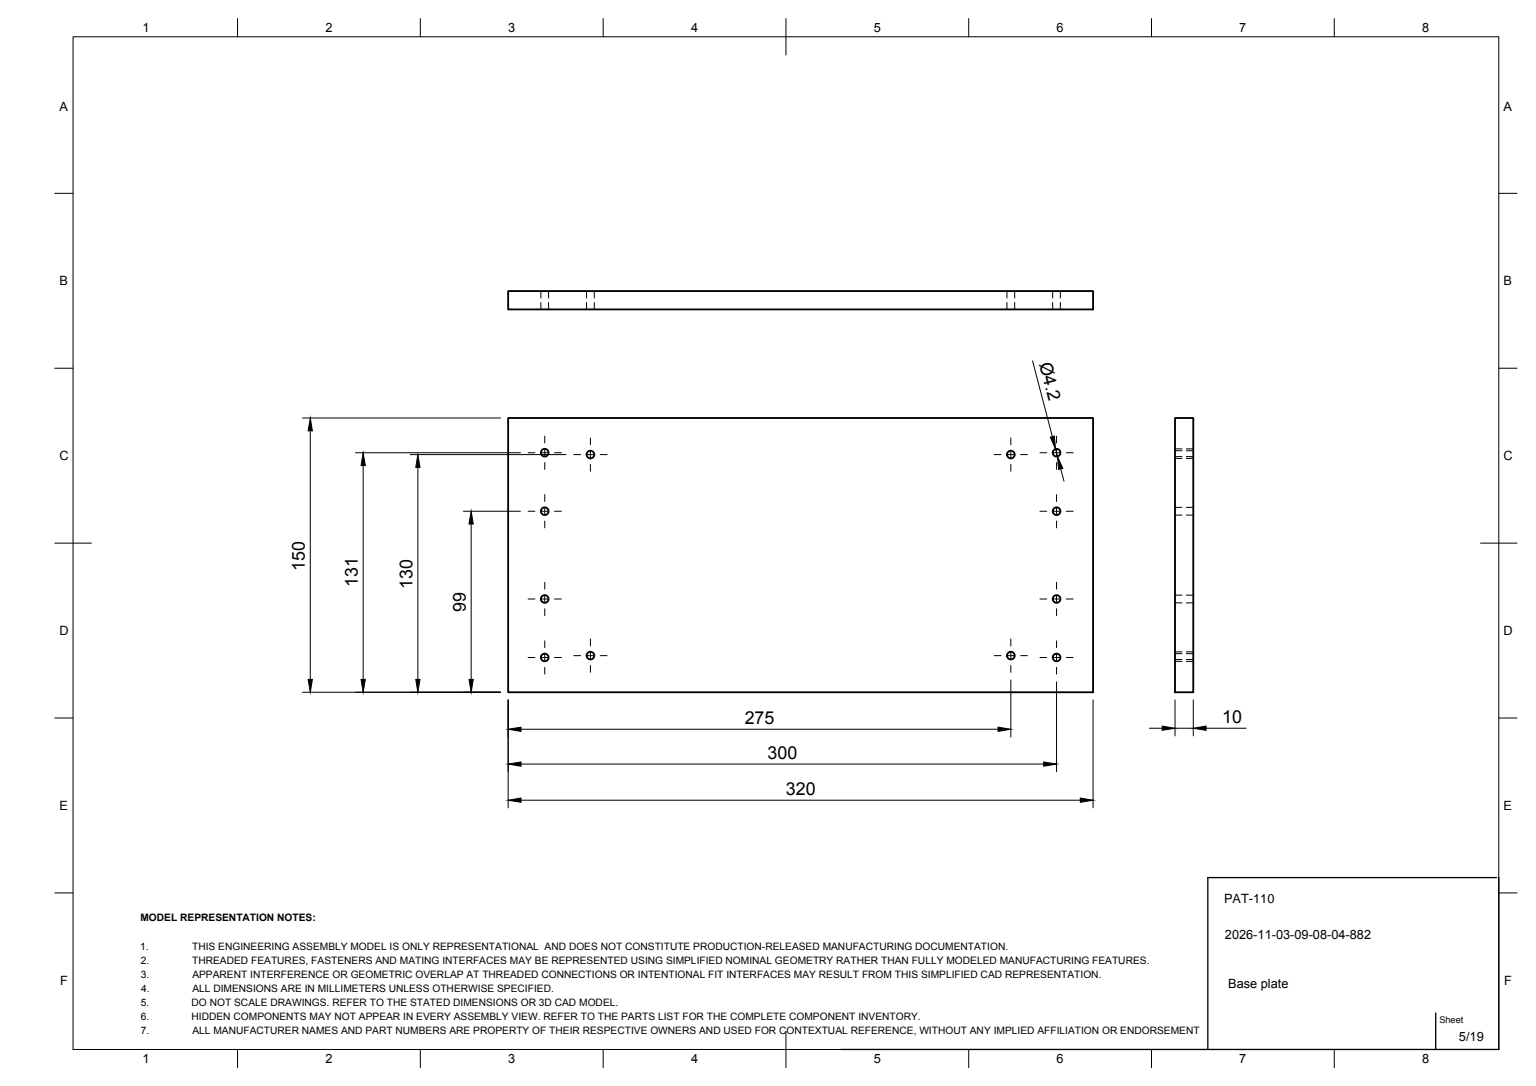
ISO-10303-21;
HEADER;
/* Generated by software containing ST-Developer
 * from STEP Tools, Inc. (www.steptools.com) 
 */

FILE_DESCRIPTION(
/* description */ ('Twin-shaft manual slide'),
/* implementation_level */ '2;1');

FILE_NAME(
/* name */ 'Base plate.step',
/* time_stamp */ '2026-10-27T18:38:08-07:00',
/* author */ (''),
/* organization */ (''),
/* preprocessor_version */ 'ST-DEVELOPER v20.2',
/* originating_system */ 'Autodesk Translation Framework v15.17.0.0',
/* authorisation */ '');

FILE_SCHEMA (('AUTOMOTIVE_DESIGN { 1 0 10303 214 3 1 1 }'));
ENDSEC;

DATA;
#10=MECHANICAL_DESIGN_GEOMETRIC_PRESENTATION_REPRESENTATION('',(#276),#6463);
#244=SHAPE_REPRESENTATION_RELATIONSHIP('SRR','None',#6562,#260);
#260=ADVANCED_BREP_SHAPE_REPRESENTATION('',(#292),#6445);
#276=STYLED_ITEM('',(#6719),#292);
#292=MANIFOLD_SOLID_BREP('Body1',#3638);
#304=FACE_BOUND('',#750,.T.);
#305=FACE_BOUND('',#751,.T.);
#306=FACE_BOUND('',#752,.T.);
#307=FACE_BOUND('',#753,.T.);
#308=FACE_BOUND('',#754,.T.);
#309=FACE_BOUND('',#755,.T.);
#310=FACE_BOUND('',#756,.T.);
#311=FACE_BOUND('',#757,.T.);
#312=FACE_BOUND('',#758,.T.);
#313=FACE_BOUND('',#759,.T.);
#314=FACE_BOUND('',#760,.T.);
#315=FACE_BOUND('',#761,.T.);
#316=FACE_BOUND('',#763,.T.);
#317=FACE_BOUND('',#764,.T.);
#318=FACE_BOUND('',#765,.T.);
#319=FACE_BOUND('',#766,.T.);
#320=FACE_BOUND('',#767,.T.);
#321=FACE_BOUND('',#768,.T.);
#322=FACE_BOUND('',#769,.T.);
#323=FACE_BOUND('',#770,.T.);
#324=FACE_BOUND('',#771,.T.);
#325=FACE_BOUND('',#772,.T.);
#326=FACE_BOUND('',#773,.T.);
#327=FACE_BOUND('',#774,.T.);
#401=PLANE('',#3874);
#402=PLANE('',#3875);
#403=PLANE('',#3876);
#404=PLANE('',#3877);
#405=PLANE('',#3878);
#406=PLANE('',#3879);
#526=FACE_OUTER_BOUND('',#733,.T.);
#527=FACE_OUTER_BOUND('',#734,.T.);
#528=FACE_OUTER_BOUND('',#735,.T.);
#529=FACE_OUTER_BOUND('',#736,.T.);
#530=FACE_OUTER_BOUND('',#737,.T.);
#531=FACE_OUTER_BOUND('',#738,.T.);
#532=FACE_OUTER_BOUND('',#739,.T.);
#533=FACE_OUTER_BOUND('',#740,.T.);
#534=FACE_OUTER_BOUND('',#741,.T.);
#535=FACE_OUTER_BOUND('',#742,.T.);
#536=FACE_OUTER_BOUND('',#743,.T.);
#537=FACE_OUTER_BOUND('',#744,.T.);
#538=FACE_OUTER_BOUND('',#745,.T.);
#539=FACE_OUTER_BOUND('',#746,.T.);
#540=FACE_OUTER_BOUND('',#747,.T.);
#541=FACE_OUTER_BOUND('',#748,.T.);
#542=FACE_OUTER_BOUND('',#749,.T.);
#543=FACE_OUTER_BOUND('',#762,.T.);
#733=EDGE_LOOP('',(#2488,#2489,#2490,#2491));
#734=EDGE_LOOP('',(#2492,#2493,#2494,#2495));
#735=EDGE_LOOP('',(#2496,#2497,#2498,#2499));
#736=EDGE_LOOP('',(#2500,#2501,#2502,#2503));
#737=EDGE_LOOP('',(#2504,#2505,#2506,#2507));
#738=EDGE_LOOP('',(#2508,#2509,#2510,#2511));
#739=EDGE_LOOP('',(#2512,#2513,#2514,#2515));
#740=EDGE_LOOP('',(#2516,#2517,#2518,#2519));
#741=EDGE_LOOP('',(#2520,#2521,#2522,#2523));
#742=EDGE_LOOP('',(#2524,#2525,#2526,#2527));
#743=EDGE_LOOP('',(#2528,#2529,#2530,#2531));
#744=EDGE_LOOP('',(#2532,#2533,#2534,#2535));
#745=EDGE_LOOP('',(#2536,#2537,#2538,#2539));
#746=EDGE_LOOP('',(#2540,#2541,#2542,#2543));
#747=EDGE_LOOP('',(#2544,#2545,#2546,#2547));
#748=EDGE_LOOP('',(#2548,#2549,#2550,#2551));
#749=EDGE_LOOP('',(#2552,#2553,#2554,#2555));
#750=EDGE_LOOP('',(#2556));
#751=EDGE_LOOP('',(#2557));
#752=EDGE_LOOP('',(#2558));
#753=EDGE_LOOP('',(#2559));
#754=EDGE_LOOP('',(#2560));
#755=EDGE_LOOP('',(#2561));
#756=EDGE_LOOP('',(#2562));
#757=EDGE_LOOP('',(#2563));
#758=EDGE_LOOP('',(#2564));
#759=EDGE_LOOP('',(#2565));
#760=EDGE_LOOP('',(#2566));
#761=EDGE_LOOP('',(#2567));
#762=EDGE_LOOP('',(#2568,#2569,#2570,#2571));
#763=EDGE_LOOP('',(#2572));
#764=EDGE_LOOP('',(#2573));
#765=EDGE_LOOP('',(#2574));
#766=EDGE_LOOP('',(#2575));
#767=EDGE_LOOP('',(#2576));
#768=EDGE_LOOP('',(#2577));
#769=EDGE_LOOP('',(#2578));
#770=EDGE_LOOP('',(#2579));
#771=EDGE_LOOP('',(#2580));
#772=EDGE_LOOP('',(#2581));
#773=EDGE_LOOP('',(#2582));
#774=EDGE_LOOP('',(#2583));
#1037=LINE('',#5424,#1323);
#1038=LINE('',#5430,#1324);
#1039=LINE('',#5436,#1325);
#1040=LINE('',#5442,#1326);
#1041=LINE('',#5448,#1327);
#1042=LINE('',#5454,#1328);
#1043=LINE('',#5460,#1329);
#1044=LINE('',#5466,#1330);
#1045=LINE('',#5472,#1331);
#1046=LINE('',#5478,#1332);
#1047=LINE('',#5484,#1333);
#1048=LINE('',#5490,#1334);
#1049=LINE('',#5495,#1335);
#1050=LINE('',#5497,#1336);
#1051=LINE('',#5499,#1337);
#1052=LINE('',#5500,#1338);
#1053=LINE('',#5503,#1339);
#1054=LINE('',#5505,#1340);
#1055=LINE('',#5506,#1341);
#1056=LINE('',#5509,#1342);
#1057=LINE('',#5511,#1343);
#1058=LINE('',#5512,#1344);
#1059=LINE('',#5514,#1345);
#1060=LINE('',#5515,#1346);
#1323=VECTOR('',#4277,0.210000000000001);
#1324=VECTOR('',#4284,0.21);
#1325=VECTOR('',#4291,0.21);
#1326=VECTOR('',#4298,0.210000000000001);
#1327=VECTOR('',#4305,0.210000000000001);
#1328=VECTOR('',#4312,0.210000000000001);
#1329=VECTOR('',#4319,0.21);
#1330=VECTOR('',#4326,0.21);
#1331=VECTOR('',#4333,0.21);
#1332=VECTOR('',#4340,0.21);
#1333=VECTOR('',#4347,0.210000000000001);
#1334=VECTOR('',#4354,0.210000000000001);
#1335=VECTOR('',#4359,1.);
#1336=VECTOR('',#4360,1.);
#1337=VECTOR('',#4361,1.);
#1338=VECTOR('',#4362,1.);
#1339=VECTOR('',#4365,1.);
#1340=VECTOR('',#4366,1.);
#1341=VECTOR('',#4367,1.);
#1342=VECTOR('',#4370,1.);
#1343=VECTOR('',#4371,1.);
#1344=VECTOR('',#4372,1.);
#1345=VECTOR('',#4375,1.);
#1346=VECTOR('',#4376,1.);
#1609=CIRCLE('',#3839,0.210000000000001);
#1610=CIRCLE('',#3840,0.210000000000001);
#1611=CIRCLE('',#3842,0.21);
#1612=CIRCLE('',#3843,0.21);
#1613=CIRCLE('',#3845,0.21);
#1614=CIRCLE('',#3846,0.21);
#1615=CIRCLE('',#3848,0.210000000000001);
#1616=CIRCLE('',#3849,0.210000000000001);
#1617=CIRCLE('',#3851,0.210000000000001);
#1618=CIRCLE('',#3852,0.210000000000001);
#1619=CIRCLE('',#3854,0.210000000000001);
#1620=CIRCLE('',#3855,0.210000000000001);
#1621=CIRCLE('',#3857,0.21);
#1622=CIRCLE('',#3858,0.21);
#1623=CIRCLE('',#3860,0.21);
#1624=CIRCLE('',#3861,0.21);
#1625=CIRCLE('',#3863,0.21);
#1626=CIRCLE('',#3864,0.21);
#1627=CIRCLE('',#3866,0.21);
#1628=CIRCLE('',#3867,0.21);
#1629=CIRCLE('',#3869,0.210000000000001);
#1630=CIRCLE('',#3870,0.210000000000001);
#1631=CIRCLE('',#3872,0.210000000000001);
#1632=CIRCLE('',#3873,0.210000000000001);
#1762=VERTEX_POINT('',#5421);
#1763=VERTEX_POINT('',#5423);
#1764=VERTEX_POINT('',#5427);
#1765=VERTEX_POINT('',#5429);
#1766=VERTEX_POINT('',#5433);
#1767=VERTEX_POINT('',#5435);
#1768=VERTEX_POINT('',#5439);
#1769=VERTEX_POINT('',#5441);
#1770=VERTEX_POINT('',#5445);
#1771=VERTEX_POINT('',#5447);
#1772=VERTEX_POINT('',#5451);
#1773=VERTEX_POINT('',#5453);
#1774=VERTEX_POINT('',#5457);
#1775=VERTEX_POINT('',#5459);
#1776=VERTEX_POINT('',#5463);
#1777=VERTEX_POINT('',#5465);
#1778=VERTEX_POINT('',#5469);
#1779=VERTEX_POINT('',#5471);
#1780=VERTEX_POINT('',#5475);
#1781=VERTEX_POINT('',#5477);
#1782=VERTEX_POINT('',#5481);
#1783=VERTEX_POINT('',#5483);
#1784=VERTEX_POINT('',#5487);
#1785=VERTEX_POINT('',#5489);
#1786=VERTEX_POINT('',#5493);
#1787=VERTEX_POINT('',#5494);
#1788=VERTEX_POINT('',#5496);
#1789=VERTEX_POINT('',#5498);
#1790=VERTEX_POINT('',#5502);
#1791=VERTEX_POINT('',#5504);
#1792=VERTEX_POINT('',#5508);
#1793=VERTEX_POINT('',#5510);
#2049=EDGE_CURVE('',#1762,#1762,#1609,.T.);
#2050=EDGE_CURVE('',#1762,#1763,#1037,.T.);
#2051=EDGE_CURVE('',#1763,#1763,#1610,.T.);
#2052=EDGE_CURVE('',#1764,#1764,#1611,.T.);
#2053=EDGE_CURVE('',#1764,#1765,#1038,.T.);
#2054=EDGE_CURVE('',#1765,#1765,#1612,.T.);
#2055=EDGE_CURVE('',#1766,#1766,#1613,.T.);
#2056=EDGE_CURVE('',#1766,#1767,#1039,.T.);
#2057=EDGE_CURVE('',#1767,#1767,#1614,.T.);
#2058=EDGE_CURVE('',#1768,#1768,#1615,.T.);
#2059=EDGE_CURVE('',#1768,#1769,#1040,.T.);
#2060=EDGE_CURVE('',#1769,#1769,#1616,.T.);
#2061=EDGE_CURVE('',#1770,#1770,#1617,.T.);
#2062=EDGE_CURVE('',#1770,#1771,#1041,.T.);
#2063=EDGE_CURVE('',#1771,#1771,#1618,.T.);
#2064=EDGE_CURVE('',#1772,#1772,#1619,.T.);
#2065=EDGE_CURVE('',#1772,#1773,#1042,.T.);
#2066=EDGE_CURVE('',#1773,#1773,#1620,.T.);
#2067=EDGE_CURVE('',#1774,#1774,#1621,.T.);
#2068=EDGE_CURVE('',#1774,#1775,#1043,.T.);
#2069=EDGE_CURVE('',#1775,#1775,#1622,.T.);
#2070=EDGE_CURVE('',#1776,#1776,#1623,.T.);
#2071=EDGE_CURVE('',#1776,#1777,#1044,.T.);
#2072=EDGE_CURVE('',#1777,#1777,#1624,.T.);
#2073=EDGE_CURVE('',#1778,#1778,#1625,.T.);
#2074=EDGE_CURVE('',#1778,#1779,#1045,.T.);
#2075=EDGE_CURVE('',#1779,#1779,#1626,.T.);
#2076=EDGE_CURVE('',#1780,#1780,#1627,.T.);
#2077=EDGE_CURVE('',#1780,#1781,#1046,.T.);
#2078=EDGE_CURVE('',#1781,#1781,#1628,.T.);
#2079=EDGE_CURVE('',#1782,#1782,#1629,.T.);
#2080=EDGE_CURVE('',#1782,#1783,#1047,.T.);
#2081=EDGE_CURVE('',#1783,#1783,#1630,.T.);
#2082=EDGE_CURVE('',#1784,#1784,#1631,.T.);
#2083=EDGE_CURVE('',#1784,#1785,#1048,.T.);
#2084=EDGE_CURVE('',#1785,#1785,#1632,.T.);
#2085=EDGE_CURVE('',#1786,#1787,#1049,.T.);
#2086=EDGE_CURVE('',#1787,#1788,#1050,.T.);
#2087=EDGE_CURVE('',#1789,#1788,#1051,.T.);
#2088=EDGE_CURVE('',#1786,#1789,#1052,.T.);
#2089=EDGE_CURVE('',#1790,#1786,#1053,.T.);
#2090=EDGE_CURVE('',#1791,#1789,#1054,.T.);
#2091=EDGE_CURVE('',#1790,#1791,#1055,.T.);
#2092=EDGE_CURVE('',#1792,#1790,#1056,.T.);
#2093=EDGE_CURVE('',#1793,#1791,#1057,.T.);
#2094=EDGE_CURVE('',#1792,#1793,#1058,.T.);
#2095=EDGE_CURVE('',#1787,#1792,#1059,.T.);
#2096=EDGE_CURVE('',#1788,#1793,#1060,.T.);
#2488=ORIENTED_EDGE('',*,*,#2049,.F.);
#2489=ORIENTED_EDGE('',*,*,#2050,.T.);
#2490=ORIENTED_EDGE('',*,*,#2051,.F.);
#2491=ORIENTED_EDGE('',*,*,#2050,.F.);
#2492=ORIENTED_EDGE('',*,*,#2052,.F.);
#2493=ORIENTED_EDGE('',*,*,#2053,.T.);
#2494=ORIENTED_EDGE('',*,*,#2054,.F.);
#2495=ORIENTED_EDGE('',*,*,#2053,.F.);
#2496=ORIENTED_EDGE('',*,*,#2055,.F.);
#2497=ORIENTED_EDGE('',*,*,#2056,.T.);
#2498=ORIENTED_EDGE('',*,*,#2057,.F.);
#2499=ORIENTED_EDGE('',*,*,#2056,.F.);
#2500=ORIENTED_EDGE('',*,*,#2058,.F.);
#2501=ORIENTED_EDGE('',*,*,#2059,.T.);
#2502=ORIENTED_EDGE('',*,*,#2060,.F.);
#2503=ORIENTED_EDGE('',*,*,#2059,.F.);
#2504=ORIENTED_EDGE('',*,*,#2061,.F.);
#2505=ORIENTED_EDGE('',*,*,#2062,.T.);
#2506=ORIENTED_EDGE('',*,*,#2063,.F.);
#2507=ORIENTED_EDGE('',*,*,#2062,.F.);
#2508=ORIENTED_EDGE('',*,*,#2064,.F.);
#2509=ORIENTED_EDGE('',*,*,#2065,.T.);
#2510=ORIENTED_EDGE('',*,*,#2066,.F.);
#2511=ORIENTED_EDGE('',*,*,#2065,.F.);
#2512=ORIENTED_EDGE('',*,*,#2067,.F.);
#2513=ORIENTED_EDGE('',*,*,#2068,.T.);
#2514=ORIENTED_EDGE('',*,*,#2069,.F.);
#2515=ORIENTED_EDGE('',*,*,#2068,.F.);
#2516=ORIENTED_EDGE('',*,*,#2070,.F.);
#2517=ORIENTED_EDGE('',*,*,#2071,.T.);
#2518=ORIENTED_EDGE('',*,*,#2072,.F.);
#2519=ORIENTED_EDGE('',*,*,#2071,.F.);
#2520=ORIENTED_EDGE('',*,*,#2073,.F.);
#2521=ORIENTED_EDGE('',*,*,#2074,.T.);
#2522=ORIENTED_EDGE('',*,*,#2075,.F.);
#2523=ORIENTED_EDGE('',*,*,#2074,.F.);
#2524=ORIENTED_EDGE('',*,*,#2076,.F.);
#2525=ORIENTED_EDGE('',*,*,#2077,.T.);
#2526=ORIENTED_EDGE('',*,*,#2078,.F.);
#2527=ORIENTED_EDGE('',*,*,#2077,.F.);
#2528=ORIENTED_EDGE('',*,*,#2079,.F.);
#2529=ORIENTED_EDGE('',*,*,#2080,.T.);
#2530=ORIENTED_EDGE('',*,*,#2081,.F.);
#2531=ORIENTED_EDGE('',*,*,#2080,.F.);
#2532=ORIENTED_EDGE('',*,*,#2082,.F.);
#2533=ORIENTED_EDGE('',*,*,#2083,.T.);
#2534=ORIENTED_EDGE('',*,*,#2084,.F.);
#2535=ORIENTED_EDGE('',*,*,#2083,.F.);
#2536=ORIENTED_EDGE('',*,*,#2085,.T.);
#2537=ORIENTED_EDGE('',*,*,#2086,.T.);
#2538=ORIENTED_EDGE('',*,*,#2087,.F.);
#2539=ORIENTED_EDGE('',*,*,#2088,.F.);
#2540=ORIENTED_EDGE('',*,*,#2089,.T.);
#2541=ORIENTED_EDGE('',*,*,#2088,.T.);
#2542=ORIENTED_EDGE('',*,*,#2090,.F.);
#2543=ORIENTED_EDGE('',*,*,#2091,.F.);
#2544=ORIENTED_EDGE('',*,*,#2092,.T.);
#2545=ORIENTED_EDGE('',*,*,#2091,.T.);
#2546=ORIENTED_EDGE('',*,*,#2093,.F.);
#2547=ORIENTED_EDGE('',*,*,#2094,.F.);
#2548=ORIENTED_EDGE('',*,*,#2095,.T.);
#2549=ORIENTED_EDGE('',*,*,#2094,.T.);
#2550=ORIENTED_EDGE('',*,*,#2096,.F.);
#2551=ORIENTED_EDGE('',*,*,#2086,.F.);
#2552=ORIENTED_EDGE('',*,*,#2096,.T.);
#2553=ORIENTED_EDGE('',*,*,#2093,.T.);
#2554=ORIENTED_EDGE('',*,*,#2090,.T.);
#2555=ORIENTED_EDGE('',*,*,#2087,.T.);
#2556=ORIENTED_EDGE('',*,*,#2063,.T.);
#2557=ORIENTED_EDGE('',*,*,#2066,.T.);
#2558=ORIENTED_EDGE('',*,*,#2069,.T.);
#2559=ORIENTED_EDGE('',*,*,#2072,.T.);
#2560=ORIENTED_EDGE('',*,*,#2075,.T.);
#2561=ORIENTED_EDGE('',*,*,#2078,.T.);
#2562=ORIENTED_EDGE('',*,*,#2081,.T.);
#2563=ORIENTED_EDGE('',*,*,#2084,.T.);
#2564=ORIENTED_EDGE('',*,*,#2060,.T.);
#2565=ORIENTED_EDGE('',*,*,#2057,.T.);
#2566=ORIENTED_EDGE('',*,*,#2054,.T.);
#2567=ORIENTED_EDGE('',*,*,#2051,.T.);
#2568=ORIENTED_EDGE('',*,*,#2095,.F.);
#2569=ORIENTED_EDGE('',*,*,#2085,.F.);
#2570=ORIENTED_EDGE('',*,*,#2089,.F.);
#2571=ORIENTED_EDGE('',*,*,#2092,.F.);
#2572=ORIENTED_EDGE('',*,*,#2061,.T.);
#2573=ORIENTED_EDGE('',*,*,#2064,.T.);
#2574=ORIENTED_EDGE('',*,*,#2067,.T.);
#2575=ORIENTED_EDGE('',*,*,#2070,.T.);
#2576=ORIENTED_EDGE('',*,*,#2073,.T.);
#2577=ORIENTED_EDGE('',*,*,#2076,.T.);
#2578=ORIENTED_EDGE('',*,*,#2079,.T.);
#2579=ORIENTED_EDGE('',*,*,#2082,.T.);
#2580=ORIENTED_EDGE('',*,*,#2058,.T.);
#2581=ORIENTED_EDGE('',*,*,#2055,.T.);
#2582=ORIENTED_EDGE('',*,*,#2052,.T.);
#2583=ORIENTED_EDGE('',*,*,#2049,.T.);
#3366=CYLINDRICAL_SURFACE('',#3838,0.210000000000001);
#3367=CYLINDRICAL_SURFACE('',#3841,0.21);
#3368=CYLINDRICAL_SURFACE('',#3844,0.21);
#3369=CYLINDRICAL_SURFACE('',#3847,0.210000000000001);
#3370=CYLINDRICAL_SURFACE('',#3850,0.210000000000001);
#3371=CYLINDRICAL_SURFACE('',#3853,0.210000000000001);
#3372=CYLINDRICAL_SURFACE('',#3856,0.21);
#3373=CYLINDRICAL_SURFACE('',#3859,0.21);
#3374=CYLINDRICAL_SURFACE('',#3862,0.21);
#3375=CYLINDRICAL_SURFACE('',#3865,0.21);
#3376=CYLINDRICAL_SURFACE('',#3868,0.210000000000001);
#3377=CYLINDRICAL_SURFACE('',#3871,0.210000000000001);
#3431=ADVANCED_FACE('',(#526),#3366,.F.);
#3432=ADVANCED_FACE('',(#527),#3367,.F.);
#3433=ADVANCED_FACE('',(#528),#3368,.F.);
#3434=ADVANCED_FACE('',(#529),#3369,.F.);
#3435=ADVANCED_FACE('',(#530),#3370,.F.);
#3436=ADVANCED_FACE('',(#531),#3371,.F.);
#3437=ADVANCED_FACE('',(#532),#3372,.F.);
#3438=ADVANCED_FACE('',(#533),#3373,.F.);
#3439=ADVANCED_FACE('',(#534),#3374,.F.);
#3440=ADVANCED_FACE('',(#535),#3375,.F.);
#3441=ADVANCED_FACE('',(#536),#3376,.F.);
#3442=ADVANCED_FACE('',(#537),#3377,.F.);
#3443=ADVANCED_FACE('',(#538),#401,.T.);
#3444=ADVANCED_FACE('',(#539),#402,.T.);
#3445=ADVANCED_FACE('',(#540),#403,.T.);
#3446=ADVANCED_FACE('',(#541),#404,.T.);
#3447=ADVANCED_FACE('',(#542,#304,#305,#306,#307,#308,#309,#310,#311,#312,
#313,#314,#315),#405,.T.);
#3448=ADVANCED_FACE('',(#543,#316,#317,#318,#319,#320,#321,#322,#323,#324,
#325,#326,#327),#406,.F.);
#3638=CLOSED_SHELL('',(#3431,#3432,#3433,#3434,#3435,#3436,#3437,#3438,
#3439,#3440,#3441,#3442,#3443,#3444,#3445,#3446,#3447,#3448));
#3837=AXIS2_PLACEMENT_3D('',#5419,#4271,#4272);
#3838=AXIS2_PLACEMENT_3D('',#5420,#4273,#4274);
#3839=AXIS2_PLACEMENT_3D('',#5422,#4275,#4276);
#3840=AXIS2_PLACEMENT_3D('',#5425,#4278,#4279);
#3841=AXIS2_PLACEMENT_3D('',#5426,#4280,#4281);
#3842=AXIS2_PLACEMENT_3D('',#5428,#4282,#4283);
#3843=AXIS2_PLACEMENT_3D('',#5431,#4285,#4286);
#3844=AXIS2_PLACEMENT_3D('',#5432,#4287,#4288);
#3845=AXIS2_PLACEMENT_3D('',#5434,#4289,#4290);
#3846=AXIS2_PLACEMENT_3D('',#5437,#4292,#4293);
#3847=AXIS2_PLACEMENT_3D('',#5438,#4294,#4295);
#3848=AXIS2_PLACEMENT_3D('',#5440,#4296,#4297);
#3849=AXIS2_PLACEMENT_3D('',#5443,#4299,#4300);
#3850=AXIS2_PLACEMENT_3D('',#5444,#4301,#4302);
#3851=AXIS2_PLACEMENT_3D('',#5446,#4303,#4304);
#3852=AXIS2_PLACEMENT_3D('',#5449,#4306,#4307);
#3853=AXIS2_PLACEMENT_3D('',#5450,#4308,#4309);
#3854=AXIS2_PLACEMENT_3D('',#5452,#4310,#4311);
#3855=AXIS2_PLACEMENT_3D('',#5455,#4313,#4314);
#3856=AXIS2_PLACEMENT_3D('',#5456,#4315,#4316);
#3857=AXIS2_PLACEMENT_3D('',#5458,#4317,#4318);
#3858=AXIS2_PLACEMENT_3D('',#5461,#4320,#4321);
#3859=AXIS2_PLACEMENT_3D('',#5462,#4322,#4323);
#3860=AXIS2_PLACEMENT_3D('',#5464,#4324,#4325);
#3861=AXIS2_PLACEMENT_3D('',#5467,#4327,#4328);
#3862=AXIS2_PLACEMENT_3D('',#5468,#4329,#4330);
#3863=AXIS2_PLACEMENT_3D('',#5470,#4331,#4332);
#3864=AXIS2_PLACEMENT_3D('',#5473,#4334,#4335);
#3865=AXIS2_PLACEMENT_3D('',#5474,#4336,#4337);
#3866=AXIS2_PLACEMENT_3D('',#5476,#4338,#4339);
#3867=AXIS2_PLACEMENT_3D('',#5479,#4341,#4342);
#3868=AXIS2_PLACEMENT_3D('',#5480,#4343,#4344);
#3869=AXIS2_PLACEMENT_3D('',#5482,#4345,#4346);
#3870=AXIS2_PLACEMENT_3D('',#5485,#4348,#4349);
#3871=AXIS2_PLACEMENT_3D('',#5486,#4350,#4351);
#3872=AXIS2_PLACEMENT_3D('',#5488,#4352,#4353);
#3873=AXIS2_PLACEMENT_3D('',#5491,#4355,#4356);
#3874=AXIS2_PLACEMENT_3D('',#5492,#4357,#4358);
#3875=AXIS2_PLACEMENT_3D('',#5501,#4363,#4364);
#3876=AXIS2_PLACEMENT_3D('',#5507,#4368,#4369);
#3877=AXIS2_PLACEMENT_3D('',#5513,#4373,#4374);
#3878=AXIS2_PLACEMENT_3D('',#5516,#4377,#4378);
#3879=AXIS2_PLACEMENT_3D('',#5517,#4379,#4380);
#4271=DIRECTION('axis',(0.,0.,1.));
#4272=DIRECTION('refdir',(1.,0.,0.));
#4273=DIRECTION('center_axis',(0.,0.,1.));
#4274=DIRECTION('ref_axis',(1.,0.,0.));
#4275=DIRECTION('center_axis',(0.,0.,1.));
#4276=DIRECTION('ref_axis',(1.,0.,0.));
#4277=DIRECTION('',(0.,0.,1.));
#4278=DIRECTION('center_axis',(0.,0.,-1.));
#4279=DIRECTION('ref_axis',(1.,0.,0.));
#4280=DIRECTION('center_axis',(0.,0.,1.));
#4281=DIRECTION('ref_axis',(1.,0.,0.));
#4282=DIRECTION('center_axis',(0.,0.,1.));
#4283=DIRECTION('ref_axis',(1.,0.,0.));
#4284=DIRECTION('',(0.,0.,1.));
#4285=DIRECTION('center_axis',(0.,0.,-1.));
#4286=DIRECTION('ref_axis',(1.,0.,0.));
#4287=DIRECTION('center_axis',(0.,0.,1.));
#4288=DIRECTION('ref_axis',(1.,0.,0.));
#4289=DIRECTION('center_axis',(0.,0.,1.));
#4290=DIRECTION('ref_axis',(1.,0.,0.));
#4291=DIRECTION('',(0.,0.,1.));
#4292=DIRECTION('center_axis',(0.,0.,-1.));
#4293=DIRECTION('ref_axis',(1.,0.,0.));
#4294=DIRECTION('center_axis',(0.,0.,1.));
#4295=DIRECTION('ref_axis',(1.,0.,0.));
#4296=DIRECTION('center_axis',(0.,0.,1.));
#4297=DIRECTION('ref_axis',(1.,0.,0.));
#4298=DIRECTION('',(0.,0.,1.));
#4299=DIRECTION('center_axis',(0.,0.,-1.));
#4300=DIRECTION('ref_axis',(1.,0.,0.));
#4301=DIRECTION('center_axis',(0.,0.,1.));
#4302=DIRECTION('ref_axis',(1.,0.,0.));
#4303=DIRECTION('center_axis',(0.,0.,1.));
#4304=DIRECTION('ref_axis',(1.,0.,0.));
#4305=DIRECTION('',(0.,0.,1.));
#4306=DIRECTION('center_axis',(0.,0.,-1.));
#4307=DIRECTION('ref_axis',(1.,0.,0.));
#4308=DIRECTION('center_axis',(0.,0.,1.));
#4309=DIRECTION('ref_axis',(1.,0.,0.));
#4310=DIRECTION('center_axis',(0.,0.,1.));
#4311=DIRECTION('ref_axis',(1.,0.,0.));
#4312=DIRECTION('',(0.,0.,1.));
#4313=DIRECTION('center_axis',(0.,0.,-1.));
#4314=DIRECTION('ref_axis',(1.,0.,0.));
#4315=DIRECTION('center_axis',(0.,0.,1.));
#4316=DIRECTION('ref_axis',(1.,0.,0.));
#4317=DIRECTION('center_axis',(0.,0.,1.));
#4318=DIRECTION('ref_axis',(1.,0.,0.));
#4319=DIRECTION('',(0.,0.,1.));
#4320=DIRECTION('center_axis',(0.,0.,-1.));
#4321=DIRECTION('ref_axis',(1.,0.,0.));
#4322=DIRECTION('center_axis',(0.,0.,1.));
#4323=DIRECTION('ref_axis',(1.,0.,0.));
#4324=DIRECTION('center_axis',(0.,0.,1.));
#4325=DIRECTION('ref_axis',(1.,0.,0.));
#4326=DIRECTION('',(0.,0.,1.));
#4327=DIRECTION('center_axis',(0.,0.,-1.));
#4328=DIRECTION('ref_axis',(1.,0.,0.));
#4329=DIRECTION('center_axis',(0.,0.,1.));
#4330=DIRECTION('ref_axis',(1.,0.,0.));
#4331=DIRECTION('center_axis',(0.,0.,1.));
#4332=DIRECTION('ref_axis',(1.,0.,0.));
#4333=DIRECTION('',(0.,0.,1.));
#4334=DIRECTION('center_axis',(0.,0.,-1.));
#4335=DIRECTION('ref_axis',(1.,0.,0.));
#4336=DIRECTION('center_axis',(0.,0.,1.));
#4337=DIRECTION('ref_axis',(1.,0.,0.));
#4338=DIRECTION('center_axis',(0.,0.,1.));
#4339=DIRECTION('ref_axis',(1.,0.,0.));
#4340=DIRECTION('',(0.,0.,1.));
#4341=DIRECTION('center_axis',(0.,0.,-1.));
#4342=DIRECTION('ref_axis',(1.,0.,0.));
#4343=DIRECTION('center_axis',(0.,0.,1.));
#4344=DIRECTION('ref_axis',(1.,0.,0.));
#4345=DIRECTION('center_axis',(0.,0.,1.));
#4346=DIRECTION('ref_axis',(1.,0.,0.));
#4347=DIRECTION('',(0.,0.,1.));
#4348=DIRECTION('center_axis',(0.,0.,-1.));
#4349=DIRECTION('ref_axis',(1.,0.,0.));
#4350=DIRECTION('center_axis',(0.,0.,1.));
#4351=DIRECTION('ref_axis',(1.,0.,0.));
#4352=DIRECTION('center_axis',(0.,0.,1.));
#4353=DIRECTION('ref_axis',(1.,0.,0.));
#4354=DIRECTION('',(0.,0.,1.));
#4355=DIRECTION('center_axis',(0.,0.,-1.));
#4356=DIRECTION('ref_axis',(1.,0.,0.));
#4357=DIRECTION('center_axis',(0.,1.,0.));
#4358=DIRECTION('ref_axis',(-1.,0.,0.));
#4359=DIRECTION('',(-1.,0.,0.));
#4360=DIRECTION('',(0.,0.,1.));
#4361=DIRECTION('',(-1.,0.,0.));
#4362=DIRECTION('',(0.,0.,1.));
#4363=DIRECTION('center_axis',(1.,0.,0.));
#4364=DIRECTION('ref_axis',(0.,1.,0.));
#4365=DIRECTION('',(0.,1.,0.));
#4366=DIRECTION('',(0.,1.,0.));
#4367=DIRECTION('',(0.,0.,1.));
#4368=DIRECTION('center_axis',(0.,-1.,0.));
#4369=DIRECTION('ref_axis',(1.,0.,0.));
#4370=DIRECTION('',(1.,0.,0.));
#4371=DIRECTION('',(1.,0.,0.));
#4372=DIRECTION('',(0.,0.,1.));
#4373=DIRECTION('center_axis',(-1.,0.,0.));
#4374=DIRECTION('ref_axis',(0.,-1.,0.));
#4375=DIRECTION('',(0.,-1.,0.));
#4376=DIRECTION('',(0.,-1.,0.));
#4377=DIRECTION('center_axis',(0.,0.,1.));
#4378=DIRECTION('ref_axis',(1.,0.,0.));
#4379=DIRECTION('center_axis',(0.,0.,1.));
#4380=DIRECTION('ref_axis',(1.,0.,0.));
#5419=CARTESIAN_POINT('',(0.,0.,0.));
#5420=CARTESIAN_POINT('Origin',(26.5,-5.5,-0.1));
#5421=CARTESIAN_POINT('',(26.29,-5.5,0.));
#5422=CARTESIAN_POINT('Origin',(26.5,-5.5,0.));
#5423=CARTESIAN_POINT('',(26.29,-5.5,1.));
#5424=CARTESIAN_POINT('',(26.29,-5.5,-0.1));
#5425=CARTESIAN_POINT('Origin',(26.5,-5.5,1.));
#5426=CARTESIAN_POINT('Origin',(3.5,5.5,-0.1));
#5427=CARTESIAN_POINT('',(3.29,5.5,0.));
#5428=CARTESIAN_POINT('Origin',(3.5,5.5,0.));
#5429=CARTESIAN_POINT('',(3.29,5.5,1.));
#5430=CARTESIAN_POINT('',(3.29,5.5,-0.1));
#5431=CARTESIAN_POINT('Origin',(3.5,5.5,1.));
#5432=CARTESIAN_POINT('Origin',(3.5,-5.5,-0.1));
#5433=CARTESIAN_POINT('',(3.29,-5.5,0.));
#5434=CARTESIAN_POINT('Origin',(3.5,-5.5,0.));
#5435=CARTESIAN_POINT('',(3.29,-5.5,1.));
#5436=CARTESIAN_POINT('',(3.29,-5.5,-0.1));
#5437=CARTESIAN_POINT('Origin',(3.5,-5.5,1.));
#5438=CARTESIAN_POINT('Origin',(26.5,5.5,-0.1));
#5439=CARTESIAN_POINT('',(26.29,5.5,0.));
#5440=CARTESIAN_POINT('Origin',(26.5,5.5,0.));
#5441=CARTESIAN_POINT('',(26.29,5.5,1.));
#5442=CARTESIAN_POINT('',(26.29,5.5,-0.1));
#5443=CARTESIAN_POINT('Origin',(26.5,5.5,1.));
#5444=CARTESIAN_POINT('Origin',(29.,2.4,-0.1));
#5445=CARTESIAN_POINT('',(28.79,2.4,0.));
#5446=CARTESIAN_POINT('Origin',(29.,2.4,0.));
#5447=CARTESIAN_POINT('',(28.79,2.4,1.));
#5448=CARTESIAN_POINT('',(28.79,2.4,-0.1));
#5449=CARTESIAN_POINT('Origin',(29.,2.4,1.));
#5450=CARTESIAN_POINT('Origin',(29.,-5.6,-0.1));
#5451=CARTESIAN_POINT('',(28.79,-5.6,0.));
#5452=CARTESIAN_POINT('Origin',(29.,-5.6,0.));
#5453=CARTESIAN_POINT('',(28.79,-5.6,1.));
#5454=CARTESIAN_POINT('',(28.79,-5.6,-0.1));
#5455=CARTESIAN_POINT('Origin',(29.,-5.6,1.));
#5456=CARTESIAN_POINT('Origin',(1.,5.6,-0.1));
#5457=CARTESIAN_POINT('',(0.79,5.6,0.));
#5458=CARTESIAN_POINT('Origin',(1.,5.6,0.));
#5459=CARTESIAN_POINT('',(0.79,5.6,1.));
#5460=CARTESIAN_POINT('',(0.79,5.6,-0.1));
#5461=CARTESIAN_POINT('Origin',(1.,5.6,1.));
#5462=CARTESIAN_POINT('Origin',(1.,-2.4,-0.1));
#5463=CARTESIAN_POINT('',(0.79,-2.4,0.));
#5464=CARTESIAN_POINT('Origin',(1.,-2.4,0.));
#5465=CARTESIAN_POINT('',(0.79,-2.4,1.));
#5466=CARTESIAN_POINT('',(0.79,-2.4,-0.1));
#5467=CARTESIAN_POINT('Origin',(1.,-2.4,1.));
#5468=CARTESIAN_POINT('Origin',(1.,2.4,-0.1));
#5469=CARTESIAN_POINT('',(0.79,2.4,0.));
#5470=CARTESIAN_POINT('Origin',(1.,2.4,0.));
#5471=CARTESIAN_POINT('',(0.79,2.4,1.));
#5472=CARTESIAN_POINT('',(0.79,2.4,-0.1));
#5473=CARTESIAN_POINT('Origin',(1.,2.4,1.));
#5474=CARTESIAN_POINT('Origin',(1.,-5.6,-0.1));
#5475=CARTESIAN_POINT('',(0.79,-5.6,0.));
#5476=CARTESIAN_POINT('Origin',(1.,-5.6,0.));
#5477=CARTESIAN_POINT('',(0.79,-5.6,1.));
#5478=CARTESIAN_POINT('',(0.79,-5.6,-0.1));
#5479=CARTESIAN_POINT('Origin',(1.,-5.6,1.));
#5480=CARTESIAN_POINT('Origin',(29.,-2.4,-0.1));
#5481=CARTESIAN_POINT('',(28.79,-2.4,0.));
#5482=CARTESIAN_POINT('Origin',(29.,-2.4,0.));
#5483=CARTESIAN_POINT('',(28.79,-2.4,1.));
#5484=CARTESIAN_POINT('',(28.79,-2.4,-0.1));
#5485=CARTESIAN_POINT('Origin',(29.,-2.4,1.));
#5486=CARTESIAN_POINT('Origin',(29.,5.6,-0.1));
#5487=CARTESIAN_POINT('',(28.79,5.6,0.));
#5488=CARTESIAN_POINT('Origin',(29.,5.6,0.));
#5489=CARTESIAN_POINT('',(28.79,5.6,1.));
#5490=CARTESIAN_POINT('',(28.79,5.6,-0.1));
#5491=CARTESIAN_POINT('Origin',(29.,5.6,1.));
#5492=CARTESIAN_POINT('Origin',(31.,7.5,0.));
#5493=CARTESIAN_POINT('',(31.,7.5,0.));
#5494=CARTESIAN_POINT('',(-1.,7.5,0.));
#5495=CARTESIAN_POINT('',(31.,7.5,0.));
#5496=CARTESIAN_POINT('',(-1.,7.5,1.));
#5497=CARTESIAN_POINT('',(-1.,7.5,0.));
#5498=CARTESIAN_POINT('',(31.,7.5,1.));
#5499=CARTESIAN_POINT('',(31.,7.5,1.));
#5500=CARTESIAN_POINT('',(31.,7.5,0.));
#5501=CARTESIAN_POINT('Origin',(31.,-7.5,0.));
#5502=CARTESIAN_POINT('',(31.,-7.5,0.));
#5503=CARTESIAN_POINT('',(31.,-7.5,0.));
#5504=CARTESIAN_POINT('',(31.,-7.5,1.));
#5505=CARTESIAN_POINT('',(31.,-7.5,1.));
#5506=CARTESIAN_POINT('',(31.,-7.5,0.));
#5507=CARTESIAN_POINT('Origin',(-1.,-7.5,0.));
#5508=CARTESIAN_POINT('',(-1.,-7.5,0.));
#5509=CARTESIAN_POINT('',(-1.,-7.5,0.));
#5510=CARTESIAN_POINT('',(-1.,-7.5,1.));
#5511=CARTESIAN_POINT('',(-1.,-7.5,1.));
#5512=CARTESIAN_POINT('',(-1.,-7.5,0.));
#5513=CARTESIAN_POINT('Origin',(-1.,7.5,0.));
#5514=CARTESIAN_POINT('',(-1.,7.5,0.));
#5515=CARTESIAN_POINT('',(-1.,7.5,1.));
#5516=CARTESIAN_POINT('Origin',(15.,0.,1.));
#5517=CARTESIAN_POINT('Origin',(15.,0.,0.));
#6424=UNCERTAINTY_MEASURE_WITH_UNIT(LENGTH_MEASURE(0.001),#6464,
'DISTANCE_ACCURACY_VALUE',
'Maximum model space distance between geometric entities at asserted c
onnectivities');
#6442=UNCERTAINTY_MEASURE_WITH_UNIT(LENGTH_MEASURE(0.001),#6464,
'DISTANCE_ACCURACY_VALUE',
'Maximum model space distance between geometric entities at asserted c
onnectivities');
#6445=(
GEOMETRIC_REPRESENTATION_CONTEXT(3)
GLOBAL_UNCERTAINTY_ASSIGNED_CONTEXT((#6424))
GLOBAL_UNIT_ASSIGNED_CONTEXT((#6464,#6466,#6467))
REPRESENTATION_CONTEXT('','3D')
);
#6463=(
GEOMETRIC_REPRESENTATION_CONTEXT(3)
GLOBAL_UNCERTAINTY_ASSIGNED_CONTEXT((#6442))
GLOBAL_UNIT_ASSIGNED_CONTEXT((#6464,#6466,#6467))
REPRESENTATION_CONTEXT('','3D')
);
#6464=(
LENGTH_UNIT()
NAMED_UNIT(*)
SI_UNIT(.CENTI.,.METRE.)
);
#6466=(
NAMED_UNIT(*)
PLANE_ANGLE_UNIT()
SI_UNIT($,.RADIAN.)
);
#6467=(
NAMED_UNIT(*)
SI_UNIT($,.STERADIAN.)
SOLID_ANGLE_UNIT()
);
#6470=SHAPE_DEFINITION_REPRESENTATION(#6490,#6562);
#6490=PRODUCT_DEFINITION_SHAPE('',$,#6583);
#6562=SHAPE_REPRESENTATION('',(#3837),#6445);
#6580=PRODUCT_DEFINITION_CONTEXT('part definition',#6642,'design');
#6583=PRODUCT_DEFINITION('Base plate','Base plate',#6603,#6580);
#6603=PRODUCT_DEFINITION_FORMATION('',$,#6646);
#6642=APPLICATION_CONTEXT(
'Core Data for Automotive Mechanical Design Process');
#6643=PRODUCT_CONTEXT('part definition',#6642,'mechanical');
#6646=PRODUCT('Base plate','Base plate','Base plate',(#6643));
#6713=COLOUR_RGB('Dark Blue',0.08,0.2,0.34);
#6714=FILL_AREA_STYLE_COLOUR('',#6713);
#6715=FILL_AREA_STYLE('',(#6714));
#6716=SURFACE_STYLE_FILL_AREA(#6715);
#6717=SURFACE_SIDE_STYLE('',(#6716));
#6718=SURFACE_STYLE_USAGE(.BOTH.,#6717);
#6719=PRESENTATION_STYLE_ASSIGNMENT((#6718));
ENDSEC;
END-ISO-10303-21;
